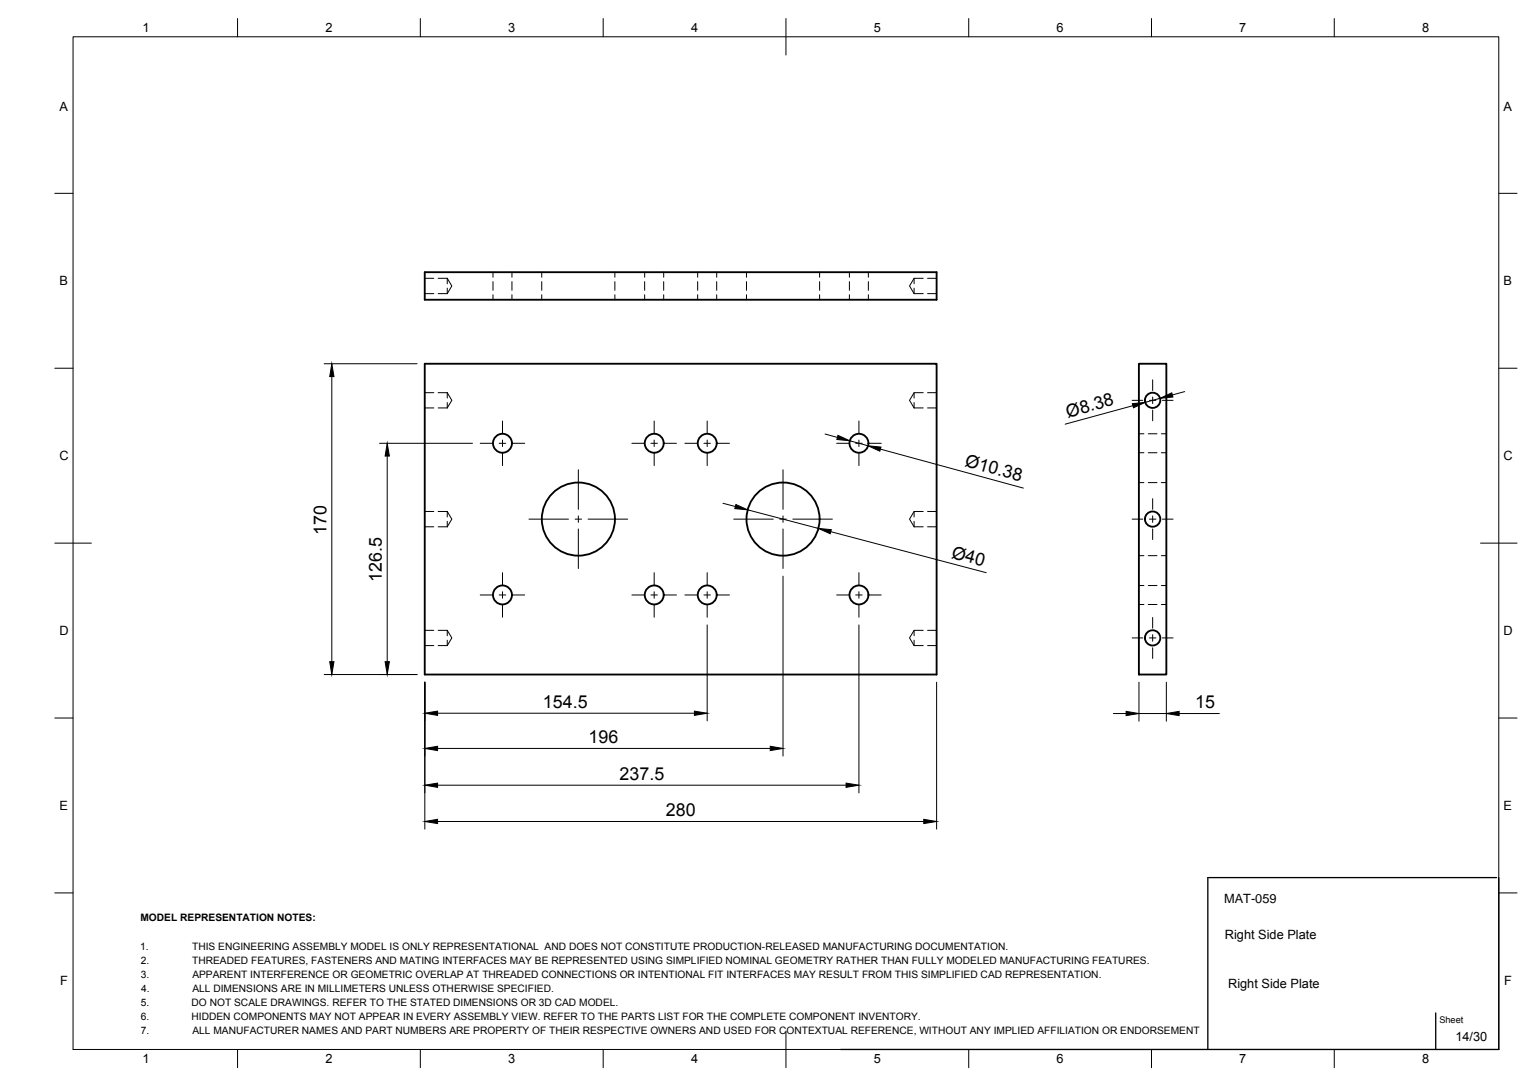
ISO-10303-21;
HEADER;
/* Generated by software containing ST-Developer
 * from STEP Tools, Inc. (www.steptools.com) 
 */

FILE_DESCRIPTION(
/* description */ ('', 'CAx-IF Rec.Pracs.---Representation and Presentation of Product Manufa
cturing Information (PMI)---4.0---2014-10-13'),
/* implementation_level */ '2;1');

FILE_NAME(
/* name */ 'Right Side Plate.step',
/* time_stamp */ '2026-10-28T23:00:48+01:00',
/* author */ (''),
/* organization */ (''),
/* preprocessor_version */ 'ST-DEVELOPER v20.2',
/* originating_system */ 'Autodesk Translation Framework v15.17.0.0',
/* authorisation */ '');

FILE_SCHEMA (('AP242_MANAGED_MODEL_BASED_3D_ENGINEERING_MIM_LF { 1 0 10303 442 2 1 4 }'));
ENDSEC;

DATA;
#10=MECHANICAL_DESIGN_GEOMETRIC_PRESENTATION_REPRESENTATION('',(#988),#61811);
#597=CONICAL_SURFACE('',#35833,2.094,1.02974425867665);
#598=CONICAL_SURFACE('',#35836,2.094,1.02974425867665);
#599=CONICAL_SURFACE('',#35839,2.094,1.02974425867665);
#600=CONICAL_SURFACE('',#35842,2.094,1.02974425867665);
#601=CONICAL_SURFACE('',#35845,2.094,1.02974425867665);
#602=CONICAL_SURFACE('',#35848,2.094,1.02974425867665);
#924=SHAPE_REPRESENTATION_RELATIONSHIP('SRR','None',#61983,#949);
#949=ADVANCED_BREP_SHAPE_REPRESENTATION('',(#1027),#61796);
#988=STYLED_ITEM('',(#62142),#1027);
#1027=MANIFOLD_SOLID_BREP('Body1',#33818);
#1343=CYLINDRICAL_SURFACE('',#35835,4.188);
#1344=CYLINDRICAL_SURFACE('',#35838,4.188);
#1345=CYLINDRICAL_SURFACE('',#35841,4.188);
#1346=CYLINDRICAL_SURFACE('',#35844,4.188);
#1347=CYLINDRICAL_SURFACE('',#35847,4.188);
#1348=CYLINDRICAL_SURFACE('',#35850,4.188);
#1349=CYLINDRICAL_SURFACE('',#35851,5.188);
#1350=CYLINDRICAL_SURFACE('',#35854,5.188);
#1351=CYLINDRICAL_SURFACE('',#35857,5.188);
#1352=CYLINDRICAL_SURFACE('',#35860,5.188);
#1353=CYLINDRICAL_SURFACE('',#35863,5.188);
#1354=CYLINDRICAL_SURFACE('',#35866,5.188);
#1355=CYLINDRICAL_SURFACE('',#35869,5.188);
#1356=CYLINDRICAL_SURFACE('',#35872,5.188);
#1357=CYLINDRICAL_SURFACE('',#35875,20.);
#1358=CYLINDRICAL_SURFACE('',#35878,20.);
#2068=FACE_BOUND('',#7199,.T.);
#2069=FACE_BOUND('',#7200,.T.);
#2070=FACE_BOUND('',#7201,.T.);
#2071=FACE_BOUND('',#7203,.T.);
#2072=FACE_BOUND('',#7204,.T.);
#2073=FACE_BOUND('',#7205,.T.);
#2074=FACE_BOUND('',#7230,.T.);
#2075=FACE_BOUND('',#7231,.T.);
#2076=FACE_BOUND('',#7232,.T.);
#2077=FACE_BOUND('',#7233,.T.);
#2078=FACE_BOUND('',#7234,.T.);
#2079=FACE_BOUND('',#7235,.T.);
#2080=FACE_BOUND('',#7236,.T.);
#2081=FACE_BOUND('',#7237,.T.);
#2082=FACE_BOUND('',#7238,.T.);
#2083=FACE_BOUND('',#7239,.T.);
#2084=FACE_BOUND('',#7242,.T.);
#2085=FACE_BOUND('',#7243,.T.);
#2086=FACE_BOUND('',#7244,.T.);
#2087=FACE_BOUND('',#7245,.T.);
#2088=FACE_BOUND('',#7246,.T.);
#2089=FACE_BOUND('',#7247,.T.);
#2090=FACE_BOUND('',#7248,.T.);
#2091=FACE_BOUND('',#7249,.T.);
#2092=FACE_BOUND('',#7250,.T.);
#2093=FACE_BOUND('',#7251,.T.);
#2984=CIRCLE('',#35825,4.188);
#2985=CIRCLE('',#35826,4.188);
#2986=CIRCLE('',#35827,4.188);
#2987=CIRCLE('',#35829,4.188);
#2988=CIRCLE('',#35830,4.188);
#2989=CIRCLE('',#35831,4.188);
#2990=CIRCLE('',#35834,4.188);
#2991=CIRCLE('',#35837,4.188);
#2992=CIRCLE('',#35840,4.188);
#2993=CIRCLE('',#35843,4.188);
#2994=CIRCLE('',#35846,4.188);
#2995=CIRCLE('',#35849,4.188);
#2996=CIRCLE('',#35852,5.188);
#2997=CIRCLE('',#35853,5.188);
#2998=CIRCLE('',#35855,5.188);
#2999=CIRCLE('',#35856,5.188);
#3000=CIRCLE('',#35858,5.188);
#3001=CIRCLE('',#35859,5.188);
#3002=CIRCLE('',#35861,5.188);
#3003=CIRCLE('',#35862,5.188);
#3004=CIRCLE('',#35864,5.188);
#3005=CIRCLE('',#35865,5.188);
#3006=CIRCLE('',#35867,5.188);
#3007=CIRCLE('',#35868,5.188);
#3008=CIRCLE('',#35870,5.188);
#3009=CIRCLE('',#35871,5.188);
#3010=CIRCLE('',#35873,5.188);
#3011=CIRCLE('',#35874,5.188);
#3012=CIRCLE('',#35876,20.);
#3013=CIRCLE('',#35877,20.);
#3014=CIRCLE('',#35879,20.);
#3015=CIRCLE('',#35880,20.);
#5130=FACE_OUTER_BOUND('',#7198,.T.);
#5131=FACE_OUTER_BOUND('',#7202,.T.);
#5132=FACE_OUTER_BOUND('',#7206,.T.);
#5133=FACE_OUTER_BOUND('',#7207,.T.);
#5134=FACE_OUTER_BOUND('',#7208,.T.);
#5135=FACE_OUTER_BOUND('',#7209,.T.);
#5136=FACE_OUTER_BOUND('',#7210,.T.);
#5137=FACE_OUTER_BOUND('',#7211,.T.);
#5138=FACE_OUTER_BOUND('',#7212,.T.);
#5139=FACE_OUTER_BOUND('',#7213,.T.);
#5140=FACE_OUTER_BOUND('',#7214,.T.);
#5141=FACE_OUTER_BOUND('',#7215,.T.);
#5142=FACE_OUTER_BOUND('',#7216,.T.);
#5143=FACE_OUTER_BOUND('',#7217,.T.);
#5144=FACE_OUTER_BOUND('',#7218,.T.);
#5145=FACE_OUTER_BOUND('',#7219,.T.);
#5146=FACE_OUTER_BOUND('',#7220,.T.);
#5147=FACE_OUTER_BOUND('',#7221,.T.);
#5148=FACE_OUTER_BOUND('',#7222,.T.);
#5149=FACE_OUTER_BOUND('',#7223,.T.);
#5150=FACE_OUTER_BOUND('',#7224,.T.);
#5151=FACE_OUTER_BOUND('',#7225,.T.);
#5152=FACE_OUTER_BOUND('',#7226,.T.);
#5153=FACE_OUTER_BOUND('',#7227,.T.);
#5154=FACE_OUTER_BOUND('',#7228,.T.);
#5155=FACE_OUTER_BOUND('',#7229,.T.);
#5156=FACE_OUTER_BOUND('',#7240,.T.);
#5157=FACE_OUTER_BOUND('',#7241,.T.);
#7198=EDGE_LOOP('',(#25930,#25931,#25932,#25933));
#7199=EDGE_LOOP('',(#25934));
#7200=EDGE_LOOP('',(#25935));
#7201=EDGE_LOOP('',(#25936));
#7202=EDGE_LOOP('',(#25937,#25938,#25939,#25940));
#7203=EDGE_LOOP('',(#25941));
#7204=EDGE_LOOP('',(#25942));
#7205=EDGE_LOOP('',(#25943));
#7206=EDGE_LOOP('',(#25944,#25945,#25946,#25947));
#7207=EDGE_LOOP('',(#25948,#25949,#25950));
#7208=EDGE_LOOP('',(#25951,#25952,#25953,#25954));
#7209=EDGE_LOOP('',(#25955,#25956,#25957));
#7210=EDGE_LOOP('',(#25958,#25959,#25960,#25961));
#7211=EDGE_LOOP('',(#25962,#25963,#25964));
#7212=EDGE_LOOP('',(#25965,#25966,#25967,#25968));
#7213=EDGE_LOOP('',(#25969,#25970,#25971));
#7214=EDGE_LOOP('',(#25972,#25973,#25974,#25975));
#7215=EDGE_LOOP('',(#25976,#25977,#25978));
#7216=EDGE_LOOP('',(#25979,#25980,#25981,#25982));
#7217=EDGE_LOOP('',(#25983,#25984,#25985));
#7218=EDGE_LOOP('',(#25986,#25987,#25988,#25989));
#7219=EDGE_LOOP('',(#25990,#25991,#25992,#25993));
#7220=EDGE_LOOP('',(#25994,#25995,#25996,#25997));
#7221=EDGE_LOOP('',(#25998,#25999,#26000,#26001));
#7222=EDGE_LOOP('',(#26002,#26003,#26004,#26005));
#7223=EDGE_LOOP('',(#26006,#26007,#26008,#26009));
#7224=EDGE_LOOP('',(#26010,#26011,#26012,#26013));
#7225=EDGE_LOOP('',(#26014,#26015,#26016,#26017));
#7226=EDGE_LOOP('',(#26018,#26019,#26020,#26021));
#7227=EDGE_LOOP('',(#26022,#26023,#26024,#26025));
#7228=EDGE_LOOP('',(#26026,#26027,#26028,#26029));
#7229=EDGE_LOOP('',(#26030,#26031,#26032,#26033));
#7230=EDGE_LOOP('',(#26034));
#7231=EDGE_LOOP('',(#26035));
#7232=EDGE_LOOP('',(#26036));
#7233=EDGE_LOOP('',(#26037));
#7234=EDGE_LOOP('',(#26038));
#7235=EDGE_LOOP('',(#26039));
#7236=EDGE_LOOP('',(#26040));
#7237=EDGE_LOOP('',(#26041));
#7238=EDGE_LOOP('',(#26042));
#7239=EDGE_LOOP('',(#26043));
#7240=EDGE_LOOP('',(#26044,#26045,#26046,#26047));
#7241=EDGE_LOOP('',(#26048,#26049,#26050,#26051));
#7242=EDGE_LOOP('',(#26052));
#7243=EDGE_LOOP('',(#26053));
#7244=EDGE_LOOP('',(#26054));
#7245=EDGE_LOOP('',(#26055));
#7246=EDGE_LOOP('',(#26056));
#7247=EDGE_LOOP('',(#26057));
#7248=EDGE_LOOP('',(#26058));
#7249=EDGE_LOOP('',(#26059));
#7250=EDGE_LOOP('',(#26060));
#7251=EDGE_LOOP('',(#26061));
#9655=LINE('',#55545,#12202);
#9656=LINE('',#55547,#12203);
#9657=LINE('',#55549,#12204);
#9658=LINE('',#55550,#12205);
#9659=LINE('',#55560,#12206);
#9660=LINE('',#55562,#12207);
#9661=LINE('',#55564,#12208);
#9662=LINE('',#55565,#12209);
#9663=LINE('',#55573,#12210);
#9664=LINE('',#55574,#12211);
#9665=LINE('',#55578,#12212);
#9666=LINE('',#55581,#12213);
#9667=LINE('',#55585,#12214);
#9668=LINE('',#55588,#12215);
#9669=LINE('',#55592,#12216);
#9670=LINE('',#55595,#12217);
#9671=LINE('',#55599,#12218);
#9672=LINE('',#55602,#12219);
#9673=LINE('',#55606,#12220);
#9674=LINE('',#55609,#12221);
#9675=LINE('',#55613,#12222);
#9676=LINE('',#55616,#12223);
#9677=LINE('',#55621,#12224);
#9678=LINE('',#55627,#12225);
#9679=LINE('',#55633,#12226);
#9680=LINE('',#55639,#12227);
#9681=LINE('',#55645,#12228);
#9682=LINE('',#55651,#12229);
#9683=LINE('',#55657,#12230);
#9684=LINE('',#55663,#12231);
#9685=LINE('',#55669,#12232);
#9686=LINE('',#55675,#12233);
#9687=LINE('',#55678,#12234);
#9688=LINE('',#55680,#12235);
#12202=VECTOR('',#42901,10.);
#12203=VECTOR('',#42902,10.);
#12204=VECTOR('',#42903,10.);
#12205=VECTOR('',#42904,10.);
#12206=VECTOR('',#42913,10.);
#12207=VECTOR('',#42914,10.);
#12208=VECTOR('',#42915,10.);
#12209=VECTOR('',#42916,10.);
#12210=VECTOR('',#42925,10.);
#12211=VECTOR('',#42926,10.);
#12212=VECTOR('',#42929,2.094);
#12213=VECTOR('',#42934,4.188);
#12214=VECTOR('',#42937,2.094);
#12215=VECTOR('',#42942,4.188);
#12216=VECTOR('',#42945,2.094);
#12217=VECTOR('',#42950,4.188);
#12218=VECTOR('',#42953,2.094);
#12219=VECTOR('',#42958,4.188);
#12220=VECTOR('',#42961,2.094);
#12221=VECTOR('',#42966,4.188);
#12222=VECTOR('',#42969,2.094);
#12223=VECTOR('',#42974,4.188);
#12224=VECTOR('',#42979,5.188);
#12225=VECTOR('',#42986,5.188);
#12226=VECTOR('',#42993,5.188);
#12227=VECTOR('',#43000,5.188);
#12228=VECTOR('',#43007,5.188);
#12229=VECTOR('',#43014,5.188);
#12230=VECTOR('',#43021,5.188);
#12231=VECTOR('',#43028,5.188);
#12232=VECTOR('',#43035,20.);
#12233=VECTOR('',#43042,20.);
#12234=VECTOR('',#43047,10.);
#12235=VECTOR('',#43050,10.);
#14896=VERTEX_POINT('',#55543);
#14897=VERTEX_POINT('',#55544);
#14898=VERTEX_POINT('',#55546);
#14899=VERTEX_POINT('',#55548);
#14900=VERTEX_POINT('',#55551);
#14901=VERTEX_POINT('',#55553);
#14902=VERTEX_POINT('',#55555);
#14903=VERTEX_POINT('',#55558);
#14904=VERTEX_POINT('',#55559);
#14905=VERTEX_POINT('',#55561);
#14906=VERTEX_POINT('',#55563);
#14907=VERTEX_POINT('',#55566);
#14908=VERTEX_POINT('',#55568);
#14909=VERTEX_POINT('',#55570);
#14910=VERTEX_POINT('',#55576);
#14911=VERTEX_POINT('',#55577);
#14912=VERTEX_POINT('',#55583);
#14913=VERTEX_POINT('',#55584);
#14914=VERTEX_POINT('',#55590);
#14915=VERTEX_POINT('',#55591);
#14916=VERTEX_POINT('',#55597);
#14917=VERTEX_POINT('',#55598);
#14918=VERTEX_POINT('',#55604);
#14919=VERTEX_POINT('',#55605);
#14920=VERTEX_POINT('',#55611);
#14921=VERTEX_POINT('',#55612);
#14922=VERTEX_POINT('',#55618);
#14923=VERTEX_POINT('',#55620);
#14924=VERTEX_POINT('',#55624);
#14925=VERTEX_POINT('',#55626);
#14926=VERTEX_POINT('',#55630);
#14927=VERTEX_POINT('',#55632);
#14928=VERTEX_POINT('',#55636);
#14929=VERTEX_POINT('',#55638);
#14930=VERTEX_POINT('',#55642);
#14931=VERTEX_POINT('',#55644);
#14932=VERTEX_POINT('',#55648);
#14933=VERTEX_POINT('',#55650);
#14934=VERTEX_POINT('',#55654);
#14935=VERTEX_POINT('',#55656);
#14936=VERTEX_POINT('',#55660);
#14937=VERTEX_POINT('',#55662);
#14938=VERTEX_POINT('',#55666);
#14939=VERTEX_POINT('',#55668);
#14940=VERTEX_POINT('',#55672);
#14941=VERTEX_POINT('',#55674);
#18867=EDGE_CURVE('',#14896,#14897,#9655,.T.);
#18868=EDGE_CURVE('',#14898,#14896,#9656,.T.);
#18869=EDGE_CURVE('',#14899,#14898,#9657,.T.);
#18870=EDGE_CURVE('',#14897,#14899,#9658,.T.);
#18871=EDGE_CURVE('',#14900,#14900,#2984,.T.);
#18872=EDGE_CURVE('',#14901,#14901,#2985,.T.);
#18873=EDGE_CURVE('',#14902,#14902,#2986,.T.);
#18874=EDGE_CURVE('',#14903,#14904,#9659,.T.);
#18875=EDGE_CURVE('',#14905,#14903,#9660,.T.);
#18876=EDGE_CURVE('',#14906,#14905,#9661,.T.);
#18877=EDGE_CURVE('',#14904,#14906,#9662,.T.);
#18878=EDGE_CURVE('',#14907,#14907,#2987,.T.);
#18879=EDGE_CURVE('',#14908,#14908,#2988,.T.);
#18880=EDGE_CURVE('',#14909,#14909,#2989,.T.);
#18881=EDGE_CURVE('',#14904,#14896,#9663,.T.);
#18882=EDGE_CURVE('',#14898,#14906,#9664,.T.);
#18883=EDGE_CURVE('',#14910,#14911,#9665,.T.);
#18884=EDGE_CURVE('',#14911,#14911,#2990,.T.);
#18885=EDGE_CURVE('',#14900,#14911,#9666,.T.);
#18886=EDGE_CURVE('',#14912,#14913,#9667,.T.);
#18887=EDGE_CURVE('',#14913,#14913,#2991,.T.);
#18888=EDGE_CURVE('',#14901,#14913,#9668,.T.);
#18889=EDGE_CURVE('',#14914,#14915,#9669,.T.);
#18890=EDGE_CURVE('',#14915,#14915,#2992,.T.);
#18891=EDGE_CURVE('',#14902,#14915,#9670,.T.);
#18892=EDGE_CURVE('',#14916,#14917,#9671,.T.);
#18893=EDGE_CURVE('',#14917,#14917,#2993,.T.);
#18894=EDGE_CURVE('',#14917,#14909,#9672,.T.);
#18895=EDGE_CURVE('',#14918,#14919,#9673,.T.);
#18896=EDGE_CURVE('',#14919,#14919,#2994,.T.);
#18897=EDGE_CURVE('',#14919,#14908,#9674,.T.);
#18898=EDGE_CURVE('',#14920,#14921,#9675,.T.);
#18899=EDGE_CURVE('',#14921,#14921,#2995,.T.);
#18900=EDGE_CURVE('',#14921,#14907,#9676,.T.);
#18901=EDGE_CURVE('',#14922,#14922,#2996,.T.);
#18902=EDGE_CURVE('',#14922,#14923,#9677,.T.);
#18903=EDGE_CURVE('',#14923,#14923,#2997,.T.);
#18904=EDGE_CURVE('',#14924,#14924,#2998,.T.);
#18905=EDGE_CURVE('',#14924,#14925,#9678,.T.);
#18906=EDGE_CURVE('',#14925,#14925,#2999,.T.);
#18907=EDGE_CURVE('',#14926,#14926,#3000,.T.);
#18908=EDGE_CURVE('',#14926,#14927,#9679,.T.);
#18909=EDGE_CURVE('',#14927,#14927,#3001,.T.);
#18910=EDGE_CURVE('',#14928,#14928,#3002,.T.);
#18911=EDGE_CURVE('',#14928,#14929,#9680,.T.);
#18912=EDGE_CURVE('',#14929,#14929,#3003,.T.);
#18913=EDGE_CURVE('',#14930,#14930,#3004,.T.);
#18914=EDGE_CURVE('',#14930,#14931,#9681,.T.);
#18915=EDGE_CURVE('',#14931,#14931,#3005,.T.);
#18916=EDGE_CURVE('',#14932,#14932,#3006,.T.);
#18917=EDGE_CURVE('',#14932,#14933,#9682,.T.);
#18918=EDGE_CURVE('',#14933,#14933,#3007,.T.);
#18919=EDGE_CURVE('',#14934,#14934,#3008,.T.);
#18920=EDGE_CURVE('',#14934,#14935,#9683,.T.);
#18921=EDGE_CURVE('',#14935,#14935,#3009,.T.);
#18922=EDGE_CURVE('',#14936,#14936,#3010,.T.);
#18923=EDGE_CURVE('',#14936,#14937,#9684,.T.);
#18924=EDGE_CURVE('',#14937,#14937,#3011,.T.);
#18925=EDGE_CURVE('',#14938,#14938,#3012,.T.);
#18926=EDGE_CURVE('',#14938,#14939,#9685,.T.);
#18927=EDGE_CURVE('',#14939,#14939,#3013,.T.);
#18928=EDGE_CURVE('',#14940,#14940,#3014,.T.);
#18929=EDGE_CURVE('',#14940,#14941,#9686,.T.);
#18930=EDGE_CURVE('',#14941,#14941,#3015,.T.);
#18931=EDGE_CURVE('',#14897,#14903,#9687,.T.);
#18932=EDGE_CURVE('',#14905,#14899,#9688,.T.);
#25930=ORIENTED_EDGE('',*,*,#18867,.F.);
#25931=ORIENTED_EDGE('',*,*,#18868,.F.);
#25932=ORIENTED_EDGE('',*,*,#18869,.F.);
#25933=ORIENTED_EDGE('',*,*,#18870,.F.);
#25934=ORIENTED_EDGE('',*,*,#18871,.F.);
#25935=ORIENTED_EDGE('',*,*,#18872,.F.);
#25936=ORIENTED_EDGE('',*,*,#18873,.F.);
#25937=ORIENTED_EDGE('',*,*,#18874,.F.);
#25938=ORIENTED_EDGE('',*,*,#18875,.F.);
#25939=ORIENTED_EDGE('',*,*,#18876,.F.);
#25940=ORIENTED_EDGE('',*,*,#18877,.F.);
#25941=ORIENTED_EDGE('',*,*,#18878,.F.);
#25942=ORIENTED_EDGE('',*,*,#18879,.F.);
#25943=ORIENTED_EDGE('',*,*,#18880,.F.);
#25944=ORIENTED_EDGE('',*,*,#18868,.T.);
#25945=ORIENTED_EDGE('',*,*,#18881,.F.);
#25946=ORIENTED_EDGE('',*,*,#18877,.T.);
#25947=ORIENTED_EDGE('',*,*,#18882,.F.);
#25948=ORIENTED_EDGE('',*,*,#18883,.T.);
#25949=ORIENTED_EDGE('',*,*,#18884,.F.);
#25950=ORIENTED_EDGE('',*,*,#18883,.F.);
#25951=ORIENTED_EDGE('',*,*,#18871,.T.);
#25952=ORIENTED_EDGE('',*,*,#18885,.T.);
#25953=ORIENTED_EDGE('',*,*,#18884,.T.);
#25954=ORIENTED_EDGE('',*,*,#18885,.F.);
#25955=ORIENTED_EDGE('',*,*,#18886,.T.);
#25956=ORIENTED_EDGE('',*,*,#18887,.F.);
#25957=ORIENTED_EDGE('',*,*,#18886,.F.);
#25958=ORIENTED_EDGE('',*,*,#18872,.T.);
#25959=ORIENTED_EDGE('',*,*,#18888,.T.);
#25960=ORIENTED_EDGE('',*,*,#18887,.T.);
#25961=ORIENTED_EDGE('',*,*,#18888,.F.);
#25962=ORIENTED_EDGE('',*,*,#18889,.T.);
#25963=ORIENTED_EDGE('',*,*,#18890,.F.);
#25964=ORIENTED_EDGE('',*,*,#18889,.F.);
#25965=ORIENTED_EDGE('',*,*,#18873,.T.);
#25966=ORIENTED_EDGE('',*,*,#18891,.T.);
#25967=ORIENTED_EDGE('',*,*,#18890,.T.);
#25968=ORIENTED_EDGE('',*,*,#18891,.F.);
#25969=ORIENTED_EDGE('',*,*,#18892,.T.);
#25970=ORIENTED_EDGE('',*,*,#18893,.T.);
#25971=ORIENTED_EDGE('',*,*,#18892,.F.);
#25972=ORIENTED_EDGE('',*,*,#18893,.F.);
#25973=ORIENTED_EDGE('',*,*,#18894,.T.);
#25974=ORIENTED_EDGE('',*,*,#18880,.T.);
#25975=ORIENTED_EDGE('',*,*,#18894,.F.);
#25976=ORIENTED_EDGE('',*,*,#18895,.T.);
#25977=ORIENTED_EDGE('',*,*,#18896,.T.);
#25978=ORIENTED_EDGE('',*,*,#18895,.F.);
#25979=ORIENTED_EDGE('',*,*,#18896,.F.);
#25980=ORIENTED_EDGE('',*,*,#18897,.T.);
#25981=ORIENTED_EDGE('',*,*,#18879,.T.);
#25982=ORIENTED_EDGE('',*,*,#18897,.F.);
#25983=ORIENTED_EDGE('',*,*,#18898,.T.);
#25984=ORIENTED_EDGE('',*,*,#18899,.T.);
#25985=ORIENTED_EDGE('',*,*,#18898,.F.);
#25986=ORIENTED_EDGE('',*,*,#18899,.F.);
#25987=ORIENTED_EDGE('',*,*,#18900,.T.);
#25988=ORIENTED_EDGE('',*,*,#18878,.T.);
#25989=ORIENTED_EDGE('',*,*,#18900,.F.);
#25990=ORIENTED_EDGE('',*,*,#18901,.F.);
#25991=ORIENTED_EDGE('',*,*,#18902,.T.);
#25992=ORIENTED_EDGE('',*,*,#18903,.F.);
#25993=ORIENTED_EDGE('',*,*,#18902,.F.);
#25994=ORIENTED_EDGE('',*,*,#18904,.F.);
#25995=ORIENTED_EDGE('',*,*,#18905,.T.);
#25996=ORIENTED_EDGE('',*,*,#18906,.F.);
#25997=ORIENTED_EDGE('',*,*,#18905,.F.);
#25998=ORIENTED_EDGE('',*,*,#18907,.F.);
#25999=ORIENTED_EDGE('',*,*,#18908,.T.);
#26000=ORIENTED_EDGE('',*,*,#18909,.F.);
#26001=ORIENTED_EDGE('',*,*,#18908,.F.);
#26002=ORIENTED_EDGE('',*,*,#18910,.F.);
#26003=ORIENTED_EDGE('',*,*,#18911,.T.);
#26004=ORIENTED_EDGE('',*,*,#18912,.F.);
#26005=ORIENTED_EDGE('',*,*,#18911,.F.);
#26006=ORIENTED_EDGE('',*,*,#18913,.F.);
#26007=ORIENTED_EDGE('',*,*,#18914,.T.);
#26008=ORIENTED_EDGE('',*,*,#18915,.F.);
#26009=ORIENTED_EDGE('',*,*,#18914,.F.);
#26010=ORIENTED_EDGE('',*,*,#18916,.F.);
#26011=ORIENTED_EDGE('',*,*,#18917,.T.);
#26012=ORIENTED_EDGE('',*,*,#18918,.F.);
#26013=ORIENTED_EDGE('',*,*,#18917,.F.);
#26014=ORIENTED_EDGE('',*,*,#18919,.F.);
#26015=ORIENTED_EDGE('',*,*,#18920,.T.);
#26016=ORIENTED_EDGE('',*,*,#18921,.F.);
#26017=ORIENTED_EDGE('',*,*,#18920,.F.);
#26018=ORIENTED_EDGE('',*,*,#18922,.F.);
#26019=ORIENTED_EDGE('',*,*,#18923,.T.);
#26020=ORIENTED_EDGE('',*,*,#18924,.F.);
#26021=ORIENTED_EDGE('',*,*,#18923,.F.);
#26022=ORIENTED_EDGE('',*,*,#18925,.F.);
#26023=ORIENTED_EDGE('',*,*,#18926,.T.);
#26024=ORIENTED_EDGE('',*,*,#18927,.F.);
#26025=ORIENTED_EDGE('',*,*,#18926,.F.);
#26026=ORIENTED_EDGE('',*,*,#18928,.F.);
#26027=ORIENTED_EDGE('',*,*,#18929,.T.);
#26028=ORIENTED_EDGE('',*,*,#18930,.F.);
#26029=ORIENTED_EDGE('',*,*,#18929,.F.);
#26030=ORIENTED_EDGE('',*,*,#18867,.T.);
#26031=ORIENTED_EDGE('',*,*,#18931,.T.);
#26032=ORIENTED_EDGE('',*,*,#18874,.T.);
#26033=ORIENTED_EDGE('',*,*,#18881,.T.);
#26034=ORIENTED_EDGE('',*,*,#18903,.T.);
#26035=ORIENTED_EDGE('',*,*,#18906,.T.);
#26036=ORIENTED_EDGE('',*,*,#18909,.T.);
#26037=ORIENTED_EDGE('',*,*,#18912,.T.);
#26038=ORIENTED_EDGE('',*,*,#18915,.T.);
#26039=ORIENTED_EDGE('',*,*,#18918,.T.);
#26040=ORIENTED_EDGE('',*,*,#18921,.T.);
#26041=ORIENTED_EDGE('',*,*,#18924,.T.);
#26042=ORIENTED_EDGE('',*,*,#18925,.T.);
#26043=ORIENTED_EDGE('',*,*,#18928,.T.);
#26044=ORIENTED_EDGE('',*,*,#18870,.T.);
#26045=ORIENTED_EDGE('',*,*,#18932,.F.);
#26046=ORIENTED_EDGE('',*,*,#18875,.T.);
#26047=ORIENTED_EDGE('',*,*,#18931,.F.);
#26048=ORIENTED_EDGE('',*,*,#18869,.T.);
#26049=ORIENTED_EDGE('',*,*,#18882,.T.);
#26050=ORIENTED_EDGE('',*,*,#18876,.T.);
#26051=ORIENTED_EDGE('',*,*,#18932,.T.);
#26052=ORIENTED_EDGE('',*,*,#18901,.T.);
#26053=ORIENTED_EDGE('',*,*,#18904,.T.);
#26054=ORIENTED_EDGE('',*,*,#18907,.T.);
#26055=ORIENTED_EDGE('',*,*,#18910,.T.);
#26056=ORIENTED_EDGE('',*,*,#18913,.T.);
#26057=ORIENTED_EDGE('',*,*,#18916,.T.);
#26058=ORIENTED_EDGE('',*,*,#18919,.T.);
#26059=ORIENTED_EDGE('',*,*,#18922,.T.);
#26060=ORIENTED_EDGE('',*,*,#18927,.T.);
#26061=ORIENTED_EDGE('',*,*,#18930,.T.);
#31594=PLANE('',#35824);
#31595=PLANE('',#35828);
#31596=PLANE('',#35832);
#31597=PLANE('',#35881);
#31598=PLANE('',#35882);
#31599=PLANE('',#35883);
#32811=ADVANCED_FACE('',(#5130,#2068,#2069,#2070),#31594,.F.);
#32812=ADVANCED_FACE('',(#5131,#2071,#2072,#2073),#31595,.F.);
#32813=ADVANCED_FACE('',(#5132),#31596,.T.);
#32814=ADVANCED_FACE('',(#5133),#597,.F.);
#32815=ADVANCED_FACE('',(#5134),#1343,.F.);
#32816=ADVANCED_FACE('',(#5135),#598,.F.);
#32817=ADVANCED_FACE('',(#5136),#1344,.F.);
#32818=ADVANCED_FACE('',(#5137),#599,.F.);
#32819=ADVANCED_FACE('',(#5138),#1345,.F.);
#32820=ADVANCED_FACE('',(#5139),#600,.F.);
#32821=ADVANCED_FACE('',(#5140),#1346,.F.);
#32822=ADVANCED_FACE('',(#5141),#601,.F.);
#32823=ADVANCED_FACE('',(#5142),#1347,.F.);
#32824=ADVANCED_FACE('',(#5143),#602,.F.);
#32825=ADVANCED_FACE('',(#5144),#1348,.F.);
#32826=ADVANCED_FACE('',(#5145),#1349,.F.);
#32827=ADVANCED_FACE('',(#5146),#1350,.F.);
#32828=ADVANCED_FACE('',(#5147),#1351,.F.);
#32829=ADVANCED_FACE('',(#5148),#1352,.F.);
#32830=ADVANCED_FACE('',(#5149),#1353,.F.);
#32831=ADVANCED_FACE('',(#5150),#1354,.F.);
#32832=ADVANCED_FACE('',(#5151),#1355,.F.);
#32833=ADVANCED_FACE('',(#5152),#1356,.F.);
#32834=ADVANCED_FACE('',(#5153),#1357,.F.);
#32835=ADVANCED_FACE('',(#5154),#1358,.F.);
#32836=ADVANCED_FACE('',(#5155,#2074,#2075,#2076,#2077,#2078,#2079,#2080,
#2081,#2082,#2083),#31597,.T.);
#32837=ADVANCED_FACE('',(#5156),#31598,.T.);
#32838=ADVANCED_FACE('',(#5157,#2084,#2085,#2086,#2087,#2088,#2089,#2090,
#2091,#2092,#2093),#31599,.T.);
#33818=CLOSED_SHELL('',(#32811,#32812,#32813,#32814,#32815,#32816,#32817,
#32818,#32819,#32820,#32821,#32822,#32823,#32824,#32825,#32826,#32827,#32828,
#32829,#32830,#32831,#32832,#32833,#32834,#32835,#32836,#32837,#32838));
#35823=AXIS2_PLACEMENT_3D('',#55541,#42897,#42898);
#35824=AXIS2_PLACEMENT_3D('',#55542,#42899,#42900);
#35825=AXIS2_PLACEMENT_3D('',#55552,#42905,#42906);
#35826=AXIS2_PLACEMENT_3D('',#55554,#42907,#42908);
#35827=AXIS2_PLACEMENT_3D('',#55556,#42909,#42910);
#35828=AXIS2_PLACEMENT_3D('',#55557,#42911,#42912);
#35829=AXIS2_PLACEMENT_3D('',#55567,#42917,#42918);
#35830=AXIS2_PLACEMENT_3D('',#55569,#42919,#42920);
#35831=AXIS2_PLACEMENT_3D('',#55571,#42921,#42922);
#35832=AXIS2_PLACEMENT_3D('',#55572,#42923,#42924);
#35833=AXIS2_PLACEMENT_3D('',#55575,#42927,#42928);
#35834=AXIS2_PLACEMENT_3D('',#55579,#42930,#42931);
#35835=AXIS2_PLACEMENT_3D('',#55580,#42932,#42933);
#35836=AXIS2_PLACEMENT_3D('',#55582,#42935,#42936);
#35837=AXIS2_PLACEMENT_3D('',#55586,#42938,#42939);
#35838=AXIS2_PLACEMENT_3D('',#55587,#42940,#42941);
#35839=AXIS2_PLACEMENT_3D('',#55589,#42943,#42944);
#35840=AXIS2_PLACEMENT_3D('',#55593,#42946,#42947);
#35841=AXIS2_PLACEMENT_3D('',#55594,#42948,#42949);
#35842=AXIS2_PLACEMENT_3D('',#55596,#42951,#42952);
#35843=AXIS2_PLACEMENT_3D('',#55600,#42954,#42955);
#35844=AXIS2_PLACEMENT_3D('',#55601,#42956,#42957);
#35845=AXIS2_PLACEMENT_3D('',#55603,#42959,#42960);
#35846=AXIS2_PLACEMENT_3D('',#55607,#42962,#42963);
#35847=AXIS2_PLACEMENT_3D('',#55608,#42964,#42965);
#35848=AXIS2_PLACEMENT_3D('',#55610,#42967,#42968);
#35849=AXIS2_PLACEMENT_3D('',#55614,#42970,#42971);
#35850=AXIS2_PLACEMENT_3D('',#55615,#42972,#42973);
#35851=AXIS2_PLACEMENT_3D('',#55617,#42975,#42976);
#35852=AXIS2_PLACEMENT_3D('',#55619,#42977,#42978);
#35853=AXIS2_PLACEMENT_3D('',#55622,#42980,#42981);
#35854=AXIS2_PLACEMENT_3D('',#55623,#42982,#42983);
#35855=AXIS2_PLACEMENT_3D('',#55625,#42984,#42985);
#35856=AXIS2_PLACEMENT_3D('',#55628,#42987,#42988);
#35857=AXIS2_PLACEMENT_3D('',#55629,#42989,#42990);
#35858=AXIS2_PLACEMENT_3D('',#55631,#42991,#42992);
#35859=AXIS2_PLACEMENT_3D('',#55634,#42994,#42995);
#35860=AXIS2_PLACEMENT_3D('',#55635,#42996,#42997);
#35861=AXIS2_PLACEMENT_3D('',#55637,#42998,#42999);
#35862=AXIS2_PLACEMENT_3D('',#55640,#43001,#43002);
#35863=AXIS2_PLACEMENT_3D('',#55641,#43003,#43004);
#35864=AXIS2_PLACEMENT_3D('',#55643,#43005,#43006);
#35865=AXIS2_PLACEMENT_3D('',#55646,#43008,#43009);
#35866=AXIS2_PLACEMENT_3D('',#55647,#43010,#43011);
#35867=AXIS2_PLACEMENT_3D('',#55649,#43012,#43013);
#35868=AXIS2_PLACEMENT_3D('',#55652,#43015,#43016);
#35869=AXIS2_PLACEMENT_3D('',#55653,#43017,#43018);
#35870=AXIS2_PLACEMENT_3D('',#55655,#43019,#43020);
#35871=AXIS2_PLACEMENT_3D('',#55658,#43022,#43023);
#35872=AXIS2_PLACEMENT_3D('',#55659,#43024,#43025);
#35873=AXIS2_PLACEMENT_3D('',#55661,#43026,#43027);
#35874=AXIS2_PLACEMENT_3D('',#55664,#43029,#43030);
#35875=AXIS2_PLACEMENT_3D('',#55665,#43031,#43032);
#35876=AXIS2_PLACEMENT_3D('',#55667,#43033,#43034);
#35877=AXIS2_PLACEMENT_3D('',#55670,#43036,#43037);
#35878=AXIS2_PLACEMENT_3D('',#55671,#43038,#43039);
#35879=AXIS2_PLACEMENT_3D('',#55673,#43040,#43041);
#35880=AXIS2_PLACEMENT_3D('',#55676,#43043,#43044);
#35881=AXIS2_PLACEMENT_3D('',#55677,#43045,#43046);
#35882=AXIS2_PLACEMENT_3D('',#55679,#43048,#43049);
#35883=AXIS2_PLACEMENT_3D('',#55681,#43051,#43052);
#42897=DIRECTION('axis',(0.,0.,1.));
#42898=DIRECTION('refdir',(1.,0.,0.));
#42899=DIRECTION('center_axis',(-1.,5.00596043934458E-16,3.99753460294061E-15));
#42900=DIRECTION('ref_axis',(-3.99753460294061E-15,2.1738969570699E-15,
-1.));
#42901=DIRECTION('',(3.99753460294061E-15,-2.1738969570699E-15,1.));
#42902=DIRECTION('',(-5.00596043934467E-16,-1.,-2.1738969570699E-15));
#42903=DIRECTION('',(-3.99753460294061E-15,2.1738969570699E-15,-1.));
#42904=DIRECTION('',(5.00596043934467E-16,1.,2.1738969570699E-15));
#42905=DIRECTION('center_axis',(1.,-5.00596043934458E-16,-3.99753460294061E-15));
#42906=DIRECTION('ref_axis',(-5.00596043934467E-16,-1.,-2.1738969570699E-15));
#42907=DIRECTION('center_axis',(1.,-5.00596043934458E-16,-3.99753460294061E-15));
#42908=DIRECTION('ref_axis',(-5.00596043934467E-16,-1.,-2.1738969570699E-15));
#42909=DIRECTION('center_axis',(1.,-5.00596043934458E-16,-3.99753460294061E-15));
#42910=DIRECTION('ref_axis',(-5.00596043934467E-16,-1.,-2.1738969570699E-15));
#42911=DIRECTION('center_axis',(1.,-5.00596043934457E-16,-4.37631657604802E-15));
#42912=DIRECTION('ref_axis',(4.37631657604802E-15,-2.1738969570699E-15,
1.));
#42913=DIRECTION('',(-4.37631657604802E-15,2.1738969570699E-15,-1.));
#42914=DIRECTION('',(-5.00596043934467E-16,-1.,-2.1738969570699E-15));
#42915=DIRECTION('',(4.37631657604802E-15,-2.1738969570699E-15,1.));
#42916=DIRECTION('',(5.00596043934467E-16,1.,2.1738969570699E-15));
#42917=DIRECTION('center_axis',(-1.,5.00596043934457E-16,4.37631657604802E-15));
#42918=DIRECTION('ref_axis',(-5.00596043934467E-16,-1.,-2.1738969570699E-15));
#42919=DIRECTION('center_axis',(-1.,5.00596043934457E-16,4.37631657604802E-15));
#42920=DIRECTION('ref_axis',(-5.00596043934467E-16,-1.,-2.1738969570699E-15));
#42921=DIRECTION('center_axis',(-1.,5.00596043934457E-16,4.37631657604802E-15));
#42922=DIRECTION('ref_axis',(-5.00596043934467E-16,-1.,-2.1738969570699E-15));
#42923=DIRECTION('center_axis',(-5.21224920635402E-15,2.1738969570699E-15,
-1.));
#42924=DIRECTION('ref_axis',(-1.,5.00596043934456E-16,5.21224920635402E-15));
#42925=DIRECTION('',(1.,-5.00596043934456E-16,-5.21224920635402E-15));
#42926=DIRECTION('',(-1.,5.00596043934456E-16,5.21224920635402E-15));
#42927=DIRECTION('center_axis',(1.,-5.00596043934456E-16,-5.21224920635402E-15));
#42928=DIRECTION('ref_axis',(-5.00596043934467E-16,-1.,-2.1738969570699E-15));
#42929=DIRECTION('',(0.515038074910054,0.857167300702112,-7.16140691382028E-16));
#42930=DIRECTION('center_axis',(-1.,5.00596043934456E-16,5.21224920635402E-15));
#42931=DIRECTION('ref_axis',(-5.00596043934467E-16,-1.,-2.1738969570699E-15));
#42932=DIRECTION('center_axis',(-1.,5.00596043934456E-16,5.21224920635402E-15));
#42933=DIRECTION('ref_axis',(-5.00596043934467E-16,-1.,-2.1738969570699E-15));
#42934=DIRECTION('',(-1.,5.00596043934456E-16,5.21224920635402E-15));
#42935=DIRECTION('center_axis',(1.,-5.00596043934456E-16,-5.21224920635402E-15));
#42936=DIRECTION('ref_axis',(-5.00596043934467E-16,-1.,-2.1738969570699E-15));
#42937=DIRECTION('',(0.515038074910054,0.857167300702112,-7.16140691382028E-16));
#42938=DIRECTION('center_axis',(-1.,5.00596043934456E-16,5.21224920635402E-15));
#42939=DIRECTION('ref_axis',(-5.00596043934467E-16,-1.,-2.1738969570699E-15));
#42940=DIRECTION('center_axis',(-1.,5.00596043934456E-16,5.21224920635402E-15));
#42941=DIRECTION('ref_axis',(-5.00596043934467E-16,-1.,-2.1738969570699E-15));
#42942=DIRECTION('',(-1.,5.00596043934456E-16,5.21224920635402E-15));
#42943=DIRECTION('center_axis',(1.,-5.00596043934456E-16,-5.21224920635402E-15));
#42944=DIRECTION('ref_axis',(-5.00596043934467E-16,-1.,-2.1738969570699E-15));
#42945=DIRECTION('',(0.515038074910054,0.857167300702112,-7.16140691382028E-16));
#42946=DIRECTION('center_axis',(-1.,5.00596043934456E-16,5.21224920635402E-15));
#42947=DIRECTION('ref_axis',(-5.00596043934467E-16,-1.,-2.1738969570699E-15));
#42948=DIRECTION('center_axis',(-1.,5.00596043934456E-16,5.21224920635402E-15));
#42949=DIRECTION('ref_axis',(-5.00596043934467E-16,-1.,-2.1738969570699E-15));
#42950=DIRECTION('',(-1.,5.00596043934456E-16,5.21224920635402E-15));
#42951=DIRECTION('center_axis',(-1.,5.00596043934456E-16,5.21224920635402E-15));
#42952=DIRECTION('ref_axis',(-5.00596043934467E-16,-1.,-2.1738969570699E-15));
#42953=DIRECTION('',(-0.515038074910054,0.857167300702113,4.44292746477431E-15));
#42954=DIRECTION('center_axis',(-1.,5.00596043934456E-16,5.21224920635402E-15));
#42955=DIRECTION('ref_axis',(-5.00596043934467E-16,-1.,-2.1738969570699E-15));
#42956=DIRECTION('center_axis',(-1.,5.00596043934456E-16,5.21224920635402E-15));
#42957=DIRECTION('ref_axis',(-5.00596043934467E-16,-1.,-2.1738969570699E-15));
#42958=DIRECTION('',(-1.,5.00596043934456E-16,5.21224920635402E-15));
#42959=DIRECTION('center_axis',(-1.,5.00596043934456E-16,5.21224920635402E-15));
#42960=DIRECTION('ref_axis',(-5.00596043934467E-16,-1.,-2.1738969570699E-15));
#42961=DIRECTION('',(-0.515038074910054,0.857167300702113,4.44292746477431E-15));
#42962=DIRECTION('center_axis',(-1.,5.00596043934456E-16,5.21224920635402E-15));
#42963=DIRECTION('ref_axis',(-5.00596043934467E-16,-1.,-2.1738969570699E-15));
#42964=DIRECTION('center_axis',(-1.,5.00596043934456E-16,5.21224920635402E-15));
#42965=DIRECTION('ref_axis',(-5.00596043934467E-16,-1.,-2.1738969570699E-15));
#42966=DIRECTION('',(-1.,5.00596043934456E-16,5.21224920635402E-15));
#42967=DIRECTION('center_axis',(-1.,5.00596043934456E-16,5.21224920635402E-15));
#42968=DIRECTION('ref_axis',(-5.00596043934467E-16,-1.,-2.1738969570699E-15));
#42969=DIRECTION('',(-0.515038074910054,0.857167300702113,4.44292746477431E-15));
#42970=DIRECTION('center_axis',(-1.,5.00596043934456E-16,5.21224920635402E-15));
#42971=DIRECTION('ref_axis',(-5.00596043934467E-16,-1.,-2.1738969570699E-15));
#42972=DIRECTION('center_axis',(-1.,5.00596043934456E-16,5.21224920635402E-15));
#42973=DIRECTION('ref_axis',(-5.00596043934467E-16,-1.,-2.1738969570699E-15));
#42974=DIRECTION('',(-1.,5.00596043934456E-16,5.21224920635402E-15));
#42975=DIRECTION('center_axis',(-5.00596043934467E-16,-1.,-2.1738969570699E-15));
#42976=DIRECTION('ref_axis',(-1.,5.00596043934456E-16,5.21224920635402E-15));
#42977=DIRECTION('center_axis',(-5.00596043934467E-16,-1.,-2.1738969570699E-15));
#42978=DIRECTION('ref_axis',(-1.,5.00596043934456E-16,5.21224920635402E-15));
#42979=DIRECTION('',(-5.00596043934467E-16,-1.,-2.1738969570699E-15));
#42980=DIRECTION('center_axis',(5.00596043934467E-16,1.,2.1738969570699E-15));
#42981=DIRECTION('ref_axis',(-1.,5.00596043934456E-16,5.21224920635402E-15));
#42982=DIRECTION('center_axis',(-5.00596043934467E-16,-1.,-2.1738969570699E-15));
#42983=DIRECTION('ref_axis',(-1.,5.00596043934456E-16,5.21224920635402E-15));
#42984=DIRECTION('center_axis',(-5.00596043934467E-16,-1.,-2.1738969570699E-15));
#42985=DIRECTION('ref_axis',(-1.,5.00596043934456E-16,5.21224920635402E-15));
#42986=DIRECTION('',(-5.00596043934467E-16,-1.,-2.1738969570699E-15));
#42987=DIRECTION('center_axis',(5.00596043934467E-16,1.,2.1738969570699E-15));
#42988=DIRECTION('ref_axis',(-1.,5.00596043934456E-16,5.21224920635402E-15));
#42989=DIRECTION('center_axis',(-5.00596043934467E-16,-1.,-2.1738969570699E-15));
#42990=DIRECTION('ref_axis',(-1.,5.00596043934456E-16,5.21224920635402E-15));
#42991=DIRECTION('center_axis',(-5.00596043934467E-16,-1.,-2.1738969570699E-15));
#42992=DIRECTION('ref_axis',(-1.,5.00596043934456E-16,5.21224920635402E-15));
#42993=DIRECTION('',(-5.00596043934467E-16,-1.,-2.1738969570699E-15));
#42994=DIRECTION('center_axis',(5.00596043934467E-16,1.,2.1738969570699E-15));
#42995=DIRECTION('ref_axis',(-1.,5.00596043934456E-16,5.21224920635402E-15));
#42996=DIRECTION('center_axis',(-5.00596043934467E-16,-1.,-2.1738969570699E-15));
#42997=DIRECTION('ref_axis',(-1.,5.00596043934456E-16,5.21224920635402E-15));
#42998=DIRECTION('center_axis',(-5.00596043934467E-16,-1.,-2.1738969570699E-15));
#42999=DIRECTION('ref_axis',(-1.,5.00596043934456E-16,5.21224920635402E-15));
#43000=DIRECTION('',(-5.00596043934467E-16,-1.,-2.1738969570699E-15));
#43001=DIRECTION('center_axis',(5.00596043934467E-16,1.,2.1738969570699E-15));
#43002=DIRECTION('ref_axis',(-1.,5.00596043934456E-16,5.21224920635402E-15));
#43003=DIRECTION('center_axis',(-5.00596043934467E-16,-1.,-2.1738969570699E-15));
#43004=DIRECTION('ref_axis',(-1.,5.00596043934456E-16,5.21224920635402E-15));
#43005=DIRECTION('center_axis',(-5.00596043934467E-16,-1.,-2.1738969570699E-15));
#43006=DIRECTION('ref_axis',(-1.,5.00596043934456E-16,5.21224920635402E-15));
#43007=DIRECTION('',(-5.00596043934467E-16,-1.,-2.1738969570699E-15));
#43008=DIRECTION('center_axis',(5.00596043934467E-16,1.,2.1738969570699E-15));
#43009=DIRECTION('ref_axis',(-1.,5.00596043934456E-16,5.21224920635402E-15));
#43010=DIRECTION('center_axis',(-5.00596043934467E-16,-1.,-2.1738969570699E-15));
#43011=DIRECTION('ref_axis',(-1.,5.00596043934456E-16,5.21224920635402E-15));
#43012=DIRECTION('center_axis',(-5.00596043934467E-16,-1.,-2.1738969570699E-15));
#43013=DIRECTION('ref_axis',(-1.,5.00596043934456E-16,5.21224920635402E-15));
#43014=DIRECTION('',(-5.00596043934467E-16,-1.,-2.1738969570699E-15));
#43015=DIRECTION('center_axis',(5.00596043934467E-16,1.,2.1738969570699E-15));
#43016=DIRECTION('ref_axis',(-1.,5.00596043934456E-16,5.21224920635402E-15));
#43017=DIRECTION('center_axis',(-5.00596043934467E-16,-1.,-2.1738969570699E-15));
#43018=DIRECTION('ref_axis',(-1.,5.00596043934456E-16,5.21224920635402E-15));
#43019=DIRECTION('center_axis',(-5.00596043934467E-16,-1.,-2.1738969570699E-15));
#43020=DIRECTION('ref_axis',(-1.,5.00596043934456E-16,5.21224920635402E-15));
#43021=DIRECTION('',(-5.00596043934467E-16,-1.,-2.1738969570699E-15));
#43022=DIRECTION('center_axis',(5.00596043934467E-16,1.,2.1738969570699E-15));
#43023=DIRECTION('ref_axis',(-1.,5.00596043934456E-16,5.21224920635402E-15));
#43024=DIRECTION('center_axis',(-5.00596043934467E-16,-1.,-2.1738969570699E-15));
#43025=DIRECTION('ref_axis',(-1.,5.00596043934456E-16,5.21224920635402E-15));
#43026=DIRECTION('center_axis',(-5.00596043934467E-16,-1.,-2.1738969570699E-15));
#43027=DIRECTION('ref_axis',(-1.,5.00596043934456E-16,5.21224920635402E-15));
#43028=DIRECTION('',(-5.00596043934467E-16,-1.,-2.1738969570699E-15));
#43029=DIRECTION('center_axis',(5.00596043934467E-16,1.,2.1738969570699E-15));
#43030=DIRECTION('ref_axis',(-1.,5.00596043934456E-16,5.21224920635402E-15));
#43031=DIRECTION('center_axis',(5.00596043934467E-16,1.,2.1738969570699E-15));
#43032=DIRECTION('ref_axis',(1.,-5.00596043934456E-16,-5.21224920635402E-15));
#43033=DIRECTION('center_axis',(5.00596043934467E-16,1.,2.1738969570699E-15));
#43034=DIRECTION('ref_axis',(1.,-5.00596043934456E-16,-5.21224920635402E-15));
#43035=DIRECTION('',(5.00596043934467E-16,1.,2.1738969570699E-15));
#43036=DIRECTION('center_axis',(-5.00596043934467E-16,-1.,-2.1738969570699E-15));
#43037=DIRECTION('ref_axis',(1.,-5.00596043934456E-16,-5.21224920635402E-15));
#43038=DIRECTION('center_axis',(5.00596043934467E-16,1.,2.1738969570699E-15));
#43039=DIRECTION('ref_axis',(1.,-5.00596043934456E-16,-5.21224920635402E-15));
#43040=DIRECTION('center_axis',(5.00596043934467E-16,1.,2.1738969570699E-15));
#43041=DIRECTION('ref_axis',(1.,-5.00596043934456E-16,-5.21224920635402E-15));
#43042=DIRECTION('',(5.00596043934467E-16,1.,2.1738969570699E-15));
#43043=DIRECTION('center_axis',(-5.00596043934467E-16,-1.,-2.1738969570699E-15));
#43044=DIRECTION('ref_axis',(1.,-5.00596043934456E-16,-5.21224920635402E-15));
#43045=DIRECTION('center_axis',(-5.00596043934467E-16,-1.,-2.1738969570699E-15));
#43046=DIRECTION('ref_axis',(1.,-5.00596043934456E-16,-5.21224920635402E-15));
#43047=DIRECTION('',(-1.,5.00596043934456E-16,5.21224920635402E-15));
#43048=DIRECTION('center_axis',(5.21224920635402E-15,-2.1738969570699E-15,
1.));
#43049=DIRECTION('ref_axis',(1.,-5.00596043934456E-16,-5.21224920635402E-15));
#43050=DIRECTION('',(1.,-5.00596043934456E-16,-5.21224920635402E-15));
#43051=DIRECTION('center_axis',(5.00596043934467E-16,1.,2.1738969570699E-15));
#43052=DIRECTION('ref_axis',(-1.,5.00596043934456E-16,5.21224920635402E-15));
#55541=CARTESIAN_POINT('',(0.,0.,0.));
#55542=CARTESIAN_POINT('Origin',(459.115917770968,-260.47200726879,530.000000551893));
#55543=CARTESIAN_POINT('',(459.115917770968,-275.47200726879,360.000000551893));
#55544=CARTESIAN_POINT('',(459.115917770968,-275.47200726879,530.000000551893));
#55545=CARTESIAN_POINT('',(459.115917770968,-275.47200726879,487.500000551892));
#55546=CARTESIAN_POINT('',(459.115917770968,-260.47200726879,360.000000551893));
#55547=CARTESIAN_POINT('',(459.115917770968,-264.22200726879,360.000000551892));
#55548=CARTESIAN_POINT('',(459.115917770968,-260.47200726879,530.000000551893));
#55549=CARTESIAN_POINT('',(459.115917770968,-260.47200726879,487.500000551892));
#55550=CARTESIAN_POINT('',(459.115917770968,-264.22200726879,530.000000551892));
#55551=CARTESIAN_POINT('',(459.115917770968,-263.78400726879,510.000000551892));
#55552=CARTESIAN_POINT('Origin',(459.115917770968,-267.97200726879,510.000000551892));
#55553=CARTESIAN_POINT('',(459.115917770968,-263.78400726879,445.000000551892));
#55554=CARTESIAN_POINT('Origin',(459.115917770968,-267.97200726879,445.000000551892));
#55555=CARTESIAN_POINT('',(459.115917770968,-263.78400726879,380.000000551892));
#55556=CARTESIAN_POINT('Origin',(459.115917770968,-267.97200726879,380.000000551892));
#55557=CARTESIAN_POINT('Origin',(179.115917770968,-260.47200726879,360.000000551894));
#55558=CARTESIAN_POINT('',(179.115917770968,-275.47200726879,530.000000551894));
#55559=CARTESIAN_POINT('',(179.115917770968,-275.47200726879,360.000000551894));
#55560=CARTESIAN_POINT('',(179.115917770968,-275.47200726879,402.500000551894));
#55561=CARTESIAN_POINT('',(179.115917770968,-260.47200726879,530.000000551894));
#55562=CARTESIAN_POINT('',(179.115917770968,-264.22200726879,530.000000551894));
#55563=CARTESIAN_POINT('',(179.115917770968,-260.47200726879,360.000000551894));
#55564=CARTESIAN_POINT('',(179.115917770968,-260.47200726879,402.500000551894));
#55565=CARTESIAN_POINT('',(179.115917770968,-264.22200726879,360.000000551894));
#55566=CARTESIAN_POINT('',(179.115917770968,-263.78400726879,380.000000551894));
#55567=CARTESIAN_POINT('Origin',(179.115917770968,-267.97200726879,380.000000551894));
#55568=CARTESIAN_POINT('',(179.115917770968,-263.78400726879,445.000000551894));
#55569=CARTESIAN_POINT('Origin',(179.115917770968,-267.97200726879,445.000000551894));
#55570=CARTESIAN_POINT('',(179.115917770968,-263.78400726879,510.000000551894));
#55571=CARTESIAN_POINT('Origin',(179.115917770968,-267.97200726879,510.000000551894));
#55572=CARTESIAN_POINT('Origin',(474.115917770967,-267.97200726879,360.000000551892));
#55573=CARTESIAN_POINT('',(164.115917770968,-275.47200726879,360.000000551894));
#55574=CARTESIAN_POINT('',(164.115917770968,-260.47200726879,360.000000551894));
#55575=CARTESIAN_POINT('Origin',(445.557715634724,-267.97200726879,510.000000551892));
#55576=CARTESIAN_POINT('',(444.299513498481,-267.97200726879,510.000000551892));
#55577=CARTESIAN_POINT('',(446.815917770968,-263.78400726879,510.000000551892));
#55578=CARTESIAN_POINT('',(445.557715634724,-265.87800726879,510.000000551892));
#55579=CARTESIAN_POINT('Origin',(446.815917770968,-267.97200726879,510.000000551892));
#55580=CARTESIAN_POINT('Origin',(460.465917770968,-267.97200726879,510.000000551892));
#55581=CARTESIAN_POINT('',(460.465917770968,-263.78400726879,510.000000551892));
#55582=CARTESIAN_POINT('Origin',(445.557715634724,-267.97200726879,445.000000551892));
#55583=CARTESIAN_POINT('',(444.29951349848,-267.97200726879,445.000000551892));
#55584=CARTESIAN_POINT('',(446.815917770968,-263.78400726879,445.000000551892));
#55585=CARTESIAN_POINT('',(445.557715634724,-265.87800726879,445.000000551892));
#55586=CARTESIAN_POINT('Origin',(446.815917770968,-267.97200726879,445.000000551892));
#55587=CARTESIAN_POINT('Origin',(460.465917770968,-267.97200726879,445.000000551892));
#55588=CARTESIAN_POINT('',(460.465917770968,-263.78400726879,445.000000551892));
#55589=CARTESIAN_POINT('Origin',(445.557715634724,-267.97200726879,380.000000551892));
#55590=CARTESIAN_POINT('',(444.29951349848,-267.97200726879,380.000000551892));
#55591=CARTESIAN_POINT('',(446.815917770968,-263.78400726879,380.000000551892));
#55592=CARTESIAN_POINT('',(445.557715634724,-265.87800726879,380.000000551892));
#55593=CARTESIAN_POINT('Origin',(446.815917770968,-267.97200726879,380.000000551892));
#55594=CARTESIAN_POINT('Origin',(460.465917770968,-267.97200726879,380.000000551892));
#55595=CARTESIAN_POINT('',(460.465917770968,-263.78400726879,380.000000551892));
#55596=CARTESIAN_POINT('Origin',(192.674119907212,-267.97200726879,510.000000551894));
#55597=CARTESIAN_POINT('',(193.932322043456,-267.97200726879,510.000000551894));
#55598=CARTESIAN_POINT('',(191.415917770968,-263.78400726879,510.000000551894));
#55599=CARTESIAN_POINT('',(192.674119907212,-265.87800726879,510.000000551894));
#55600=CARTESIAN_POINT('Origin',(191.415917770968,-267.97200726879,510.000000551894));
#55601=CARTESIAN_POINT('Origin',(177.765917770968,-267.97200726879,510.000000551894));
#55602=CARTESIAN_POINT('',(177.765917770968,-263.78400726879,510.000000551894));
#55603=CARTESIAN_POINT('Origin',(192.674119907212,-267.97200726879,445.000000551894));
#55604=CARTESIAN_POINT('',(193.932322043456,-267.97200726879,445.000000551894));
#55605=CARTESIAN_POINT('',(191.415917770968,-263.78400726879,445.000000551894));
#55606=CARTESIAN_POINT('',(192.674119907212,-265.87800726879,445.000000551894));
#55607=CARTESIAN_POINT('Origin',(191.415917770968,-267.97200726879,445.000000551894));
#55608=CARTESIAN_POINT('Origin',(177.765917770968,-267.97200726879,445.000000551894));
#55609=CARTESIAN_POINT('',(177.765917770968,-263.78400726879,445.000000551894));
#55610=CARTESIAN_POINT('Origin',(192.674119907212,-267.97200726879,380.000000551894));
#55611=CARTESIAN_POINT('',(193.932322043455,-267.97200726879,380.000000551894));
#55612=CARTESIAN_POINT('',(191.415917770968,-263.78400726879,380.000000551894));
#55613=CARTESIAN_POINT('',(192.674119907212,-265.87800726879,380.000000551894));
#55614=CARTESIAN_POINT('Origin',(191.415917770968,-267.97200726879,380.000000551894));
#55615=CARTESIAN_POINT('Origin',(177.765917770968,-267.97200726879,380.000000551894));
#55616=CARTESIAN_POINT('',(177.765917770968,-263.78400726879,380.000000551894));
#55617=CARTESIAN_POINT('Origin',(221.615917770968,-259.82200726879,486.500000551893));
#55618=CARTESIAN_POINT('',(226.803917770968,-260.47200726879,486.500000551893));
#55619=CARTESIAN_POINT('Origin',(221.615917770968,-260.47200726879,486.500000551893));
#55620=CARTESIAN_POINT('',(226.803917770968,-275.47200726879,486.500000551893));
#55621=CARTESIAN_POINT('',(226.803917770968,-259.82200726879,486.500000551893));
#55622=CARTESIAN_POINT('Origin',(221.615917770968,-275.47200726879,486.500000551893));
#55623=CARTESIAN_POINT('Origin',(333.615917770968,-259.82200726879,403.500000551893));
#55624=CARTESIAN_POINT('',(338.803917770968,-260.47200726879,403.500000551893));
#55625=CARTESIAN_POINT('Origin',(333.615917770968,-260.47200726879,403.500000551893));
#55626=CARTESIAN_POINT('',(338.803917770968,-275.47200726879,403.500000551893));
#55627=CARTESIAN_POINT('',(338.803917770968,-259.82200726879,403.500000551893));
#55628=CARTESIAN_POINT('Origin',(333.615917770968,-275.47200726879,403.500000551893));
#55629=CARTESIAN_POINT('Origin',(333.615917770968,-259.82200726879,486.500000551893));
#55630=CARTESIAN_POINT('',(338.803917770968,-260.47200726879,486.500000551893));
#55631=CARTESIAN_POINT('Origin',(333.615917770968,-260.47200726879,486.500000551893));
#55632=CARTESIAN_POINT('',(338.803917770968,-275.47200726879,486.500000551893));
#55633=CARTESIAN_POINT('',(338.803917770968,-259.82200726879,486.500000551893));
#55634=CARTESIAN_POINT('Origin',(333.615917770968,-275.47200726879,486.500000551893));
#55635=CARTESIAN_POINT('Origin',(416.615917770968,-259.82200726879,486.500000551892));
#55636=CARTESIAN_POINT('',(421.803917770968,-260.47200726879,486.500000551892));
#55637=CARTESIAN_POINT('Origin',(416.615917770968,-260.47200726879,486.500000551892));
#55638=CARTESIAN_POINT('',(421.803917770968,-275.47200726879,486.500000551892));
#55639=CARTESIAN_POINT('',(421.803917770968,-259.82200726879,486.500000551892));
#55640=CARTESIAN_POINT('Origin',(416.615917770968,-275.47200726879,486.500000551892));
#55641=CARTESIAN_POINT('Origin',(416.615917770968,-259.82200726879,403.500000551892));
#55642=CARTESIAN_POINT('',(421.803917770968,-260.47200726879,403.500000551892));
#55643=CARTESIAN_POINT('Origin',(416.615917770968,-260.47200726879,403.500000551892));
#55644=CARTESIAN_POINT('',(421.803917770968,-275.47200726879,403.500000551892));
#55645=CARTESIAN_POINT('',(421.803917770968,-259.82200726879,403.500000551892));
#55646=CARTESIAN_POINT('Origin',(416.615917770968,-275.47200726879,403.500000551892));
#55647=CARTESIAN_POINT('Origin',(304.615917770968,-259.82200726879,486.500000551893));
#55648=CARTESIAN_POINT('',(309.803917770968,-260.47200726879,486.500000551893));
#55649=CARTESIAN_POINT('Origin',(304.615917770968,-260.47200726879,486.500000551893));
#55650=CARTESIAN_POINT('',(309.803917770968,-275.47200726879,486.500000551893));
#55651=CARTESIAN_POINT('',(309.803917770968,-259.82200726879,486.500000551893));
#55652=CARTESIAN_POINT('Origin',(304.615917770968,-275.47200726879,486.500000551893));
#55653=CARTESIAN_POINT('Origin',(304.615917770968,-259.82200726879,403.500000551893));
#55654=CARTESIAN_POINT('',(309.803917770968,-260.47200726879,403.500000551893));
#55655=CARTESIAN_POINT('Origin',(304.615917770968,-260.47200726879,403.500000551893));
#55656=CARTESIAN_POINT('',(309.803917770968,-275.47200726879,403.500000551893));
#55657=CARTESIAN_POINT('',(309.803917770968,-259.82200726879,403.500000551893));
#55658=CARTESIAN_POINT('Origin',(304.615917770968,-275.47200726879,403.500000551893));
#55659=CARTESIAN_POINT('Origin',(221.615917770968,-259.82200726879,403.500000551893));
#55660=CARTESIAN_POINT('',(226.803917770968,-260.47200726879,403.500000551893));
#55661=CARTESIAN_POINT('Origin',(221.615917770968,-260.47200726879,403.500000551893));
#55662=CARTESIAN_POINT('',(226.803917770968,-275.47200726879,403.500000551893));
#55663=CARTESIAN_POINT('',(226.803917770968,-259.82200726879,403.500000551893));
#55664=CARTESIAN_POINT('Origin',(221.615917770968,-275.47200726879,403.500000551893));
#55665=CARTESIAN_POINT('Origin',(375.115917770968,-275.47200726879,445.000000551892));
#55666=CARTESIAN_POINT('',(355.115917770968,-275.47200726879,445.000000551892));
#55667=CARTESIAN_POINT('Origin',(375.115917770968,-275.47200726879,445.000000551892));
#55668=CARTESIAN_POINT('',(355.115917770968,-260.47200726879,445.000000551892));
#55669=CARTESIAN_POINT('',(355.115917770968,-275.47200726879,445.000000551892));
#55670=CARTESIAN_POINT('Origin',(375.115917770968,-260.47200726879,445.000000551892));
#55671=CARTESIAN_POINT('Origin',(263.115917770968,-275.47200726879,445.000000551893));
#55672=CARTESIAN_POINT('',(243.115917770968,-275.47200726879,445.000000551893));
#55673=CARTESIAN_POINT('Origin',(263.115917770968,-275.47200726879,445.000000551893));
#55674=CARTESIAN_POINT('',(243.115917770968,-260.47200726879,445.000000551893));
#55675=CARTESIAN_POINT('',(243.115917770968,-275.47200726879,445.000000551893));
#55676=CARTESIAN_POINT('Origin',(263.115917770968,-260.47200726879,445.000000551893));
#55677=CARTESIAN_POINT('Origin',(319.115917770968,-275.47200726879,445.000000551893));
#55678=CARTESIAN_POINT('',(474.115917770968,-275.47200726879,530.000000551892));
#55679=CARTESIAN_POINT('Origin',(164.115917770968,-267.97200726879,530.000000551894));
#55680=CARTESIAN_POINT('',(474.115917770968,-260.47200726879,530.000000551892));
#55681=CARTESIAN_POINT('Origin',(319.115917770968,-260.47200726879,445.000000551893));
#61765=UNCERTAINTY_MEASURE_WITH_UNIT(LENGTH_MEASURE(0.01),#61812,
'DISTANCE_ACCURACY_VALUE',
'Maximum model space distance between geometric entities at asserted c
onnectivities');
#61780=UNCERTAINTY_MEASURE_WITH_UNIT(LENGTH_MEASURE(0.01),#61812,
'DISTANCE_ACCURACY_VALUE',
'Maximum model space distance between geometric entities at asserted c
onnectivities');
#61796=(
GEOMETRIC_REPRESENTATION_CONTEXT(3)
GLOBAL_UNCERTAINTY_ASSIGNED_CONTEXT((#61765))
GLOBAL_UNIT_ASSIGNED_CONTEXT((#61812,#61814,#61815))
REPRESENTATION_CONTEXT('','3D')
);
#61811=(
GEOMETRIC_REPRESENTATION_CONTEXT(3)
GLOBAL_UNCERTAINTY_ASSIGNED_CONTEXT((#61780))
GLOBAL_UNIT_ASSIGNED_CONTEXT((#61812,#61814,#61815))
REPRESENTATION_CONTEXT('','3D')
);
#61812=(
LENGTH_UNIT()
NAMED_UNIT(*)
SI_UNIT(.MILLI.,.METRE.)
);
#61814=(
NAMED_UNIT(*)
PLANE_ANGLE_UNIT()
SI_UNIT($,.RADIAN.)
);
#61815=(
NAMED_UNIT(*)
SI_UNIT($,.STERADIAN.)
SOLID_ANGLE_UNIT()
);
#61831=SHAPE_DEFINITION_REPRESENTATION(#61861,#61983);
#61861=PRODUCT_DEFINITION_SHAPE('',$,#62014);
#61983=SHAPE_REPRESENTATION('',(#35823),#61796);
#61998=PRODUCT_DEFINITION_CONTEXT('part definition',#62090,'design');
#62014=PRODUCT_DEFINITION('Right Side Plate','Right Side Plate',#62044,
#61998);
#62044=PRODUCT_DEFINITION_FORMATION('',$,#62107);
#62090=APPLICATION_CONTEXT('Managed model based 3d engineering');
#62091=PRODUCT_CONTEXT('part definition',#62090,'mechanical');
#62107=PRODUCT('Right Side Plate','Right Side Plate',$,(#62091));
#62136=COLOUR_RGB('Light Blue',0.38,0.62,0.78);
#62137=FILL_AREA_STYLE_COLOUR('',#62136);
#62138=FILL_AREA_STYLE('',(#62137));
#62139=SURFACE_STYLE_FILL_AREA(#62138);
#62140=SURFACE_SIDE_STYLE('',(#62139));
#62141=SURFACE_STYLE_USAGE(.BOTH.,#62140);
#62142=PRESENTATION_STYLE_ASSIGNMENT((#62141));
ENDSEC;
END-ISO-10303-21;
